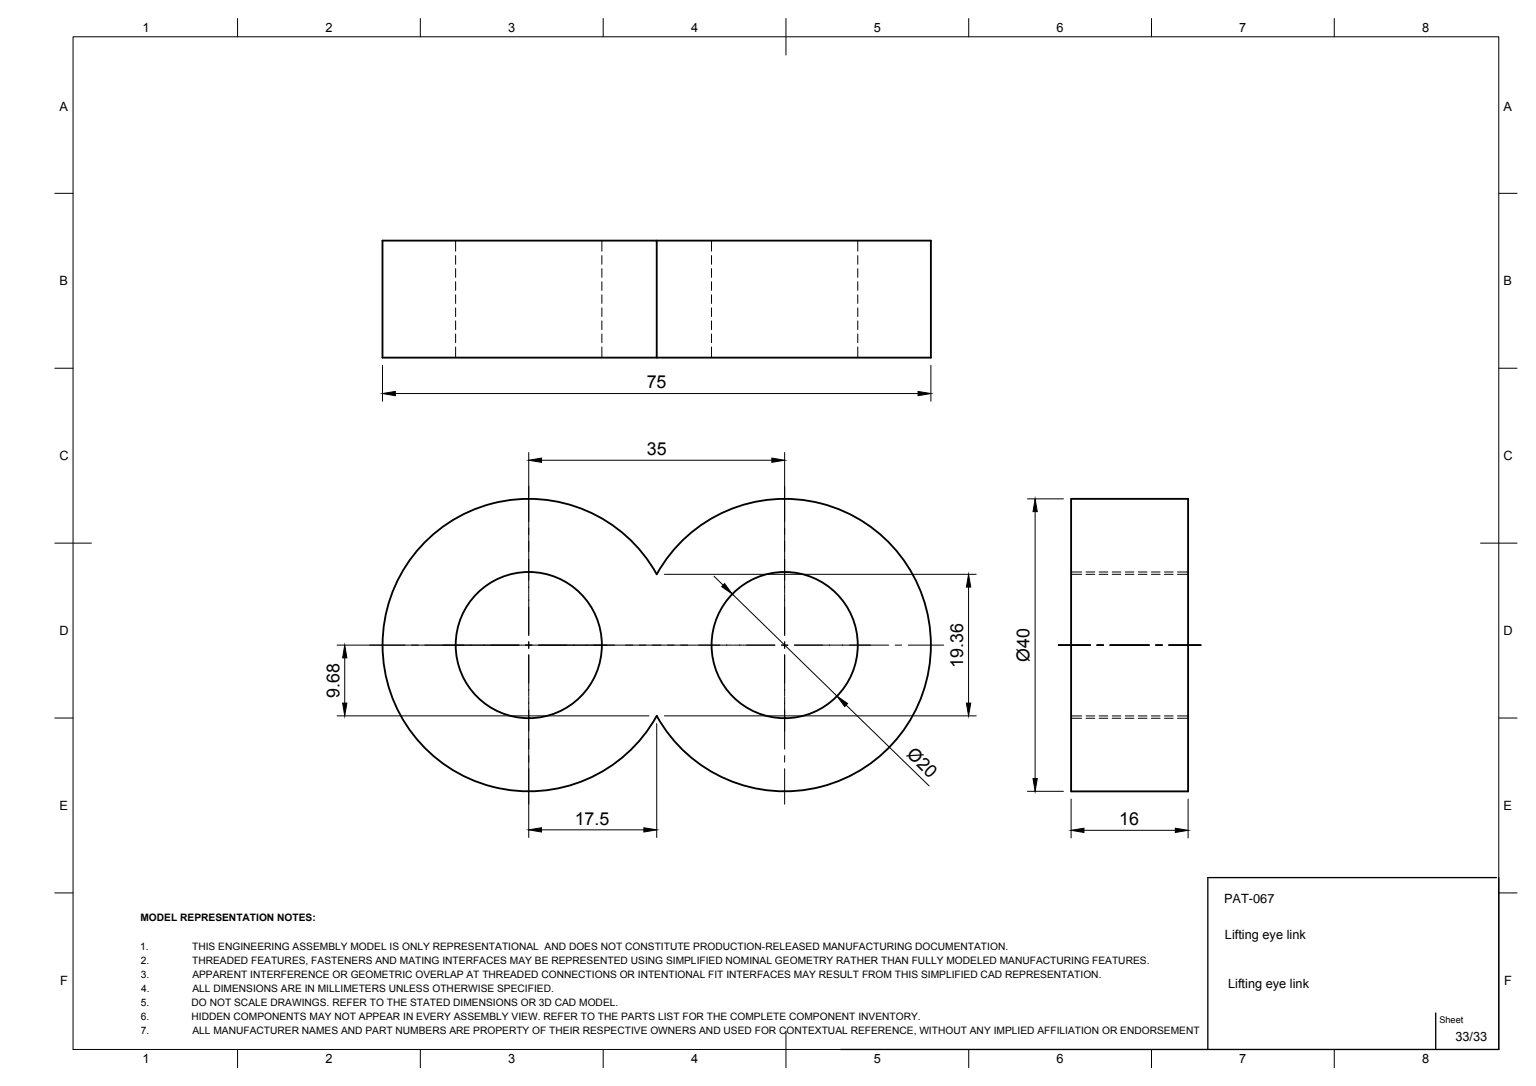
ISO-10303-21;
HEADER;
/* Generated by software containing ST-Developer
 * from STEP Tools, Inc. (www.steptools.com) 
 */

FILE_DESCRIPTION(
/* description */ ('Lifting hook block with sheave'),
/* implementation_level */ '2;1');

FILE_NAME(
/* name */ 'Lifting eye link.step',
/* time_stamp */ '2026-10-28T03:23:54-07:00',
/* author */ (''),
/* organization */ (''),
/* preprocessor_version */ 'ST-DEVELOPER v20.2',
/* originating_system */ 'Autodesk Translation Framework v15.17.0.0',
/* authorisation */ '');

FILE_SCHEMA (('AUTOMOTIVE_DESIGN { 1 0 10303 214 3 1 1 }'));
ENDSEC;

DATA;
#10=MECHANICAL_DESIGN_GEOMETRIC_PRESENTATION_REPRESENTATION('',(#388),#9391);
#320=SHAPE_REPRESENTATION_RELATIONSHIP('SRR','None',#9555,#350);
#350=ADVANCED_BREP_SHAPE_REPRESENTATION('',(#423),#9390);
#388=STYLED_ITEM('',(#9752),#423);
#423=MANIFOLD_SOLID_BREP('Body1',#4927);
#708=LINE('',#9291,#996);
#709=LINE('',#9297,#997);
#710=LINE('',#9302,#998);
#711=LINE('',#9306,#999);
#996=VECTOR('',#7519,1.);
#997=VECTOR('',#7526,1.);
#998=VECTOR('',#7531,1.);
#999=VECTOR('',#7534,1.);
#1103=CYLINDRICAL_SURFACE('',#5910,1.);
#1104=CYLINDRICAL_SURFACE('',#5913,1.);
#1105=CYLINDRICAL_SURFACE('',#5916,2.);
#1106=CYLINDRICAL_SURFACE('',#5921,2.);
#1218=FACE_BOUND('',#1909,.T.);
#1219=FACE_BOUND('',#1910,.T.);
#1220=FACE_BOUND('',#1913,.T.);
#1221=FACE_BOUND('',#1914,.T.);
#1505=FACE_OUTER_BOUND('',#1905,.T.);
#1506=FACE_OUTER_BOUND('',#1906,.T.);
#1507=FACE_OUTER_BOUND('',#1907,.T.);
#1508=FACE_OUTER_BOUND('',#1908,.T.);
#1509=FACE_OUTER_BOUND('',#1911,.T.);
#1510=FACE_OUTER_BOUND('',#1912,.T.);
#1905=EDGE_LOOP('',(#4428,#4429,#4430,#4431));
#1906=EDGE_LOOP('',(#4432,#4433,#4434,#4435));
#1907=EDGE_LOOP('',(#4436,#4437,#4438,#4439));
#1908=EDGE_LOOP('',(#4440,#4441));
#1909=EDGE_LOOP('',(#4442));
#1910=EDGE_LOOP('',(#4443));
#1911=EDGE_LOOP('',(#4444,#4445,#4446,#4447));
#1912=EDGE_LOOP('',(#4448,#4449));
#1913=EDGE_LOOP('',(#4450));
#1914=EDGE_LOOP('',(#4451));
#2200=CIRCLE('',#5911,1.);
#2201=CIRCLE('',#5912,1.);
#2202=CIRCLE('',#5914,1.);
#2203=CIRCLE('',#5915,1.);
#2204=CIRCLE('',#5917,2.);
#2205=CIRCLE('',#5918,2.);
#2206=CIRCLE('',#5920,2.);
#2207=CIRCLE('',#5922,2.);
#2611=VERTEX_POINT('',#9288);
#2612=VERTEX_POINT('',#9290);
#2613=VERTEX_POINT('',#9294);
#2614=VERTEX_POINT('',#9296);
#2615=VERTEX_POINT('',#9300);
#2616=VERTEX_POINT('',#9301);
#2617=VERTEX_POINT('',#9303);
#2618=VERTEX_POINT('',#9305);
#3218=EDGE_CURVE('',#2611,#2611,#2200,.T.);
#3219=EDGE_CURVE('',#2611,#2612,#708,.T.);
#3220=EDGE_CURVE('',#2612,#2612,#2201,.T.);
#3221=EDGE_CURVE('',#2613,#2613,#2202,.T.);
#3222=EDGE_CURVE('',#2613,#2614,#709,.T.);
#3223=EDGE_CURVE('',#2614,#2614,#2203,.T.);
#3224=EDGE_CURVE('',#2615,#2616,#710,.T.);
#3225=EDGE_CURVE('',#2615,#2617,#2204,.T.);
#3226=EDGE_CURVE('',#2618,#2617,#711,.T.);
#3227=EDGE_CURVE('',#2616,#2618,#2205,.T.);
#3228=EDGE_CURVE('',#2618,#2616,#2206,.T.);
#3229=EDGE_CURVE('',#2617,#2615,#2207,.T.);
#4428=ORIENTED_EDGE('',*,*,#3218,.F.);
#4429=ORIENTED_EDGE('',*,*,#3219,.T.);
#4430=ORIENTED_EDGE('',*,*,#3220,.F.);
#4431=ORIENTED_EDGE('',*,*,#3219,.F.);
#4432=ORIENTED_EDGE('',*,*,#3221,.F.);
#4433=ORIENTED_EDGE('',*,*,#3222,.T.);
#4434=ORIENTED_EDGE('',*,*,#3223,.F.);
#4435=ORIENTED_EDGE('',*,*,#3222,.F.);
#4436=ORIENTED_EDGE('',*,*,#3224,.F.);
#4437=ORIENTED_EDGE('',*,*,#3225,.T.);
#4438=ORIENTED_EDGE('',*,*,#3226,.F.);
#4439=ORIENTED_EDGE('',*,*,#3227,.F.);
#4440=ORIENTED_EDGE('',*,*,#3228,.T.);
#4441=ORIENTED_EDGE('',*,*,#3227,.T.);
#4442=ORIENTED_EDGE('',*,*,#3220,.T.);
#4443=ORIENTED_EDGE('',*,*,#3223,.T.);
#4444=ORIENTED_EDGE('',*,*,#3224,.T.);
#4445=ORIENTED_EDGE('',*,*,#3228,.F.);
#4446=ORIENTED_EDGE('',*,*,#3226,.T.);
#4447=ORIENTED_EDGE('',*,*,#3229,.T.);
#4448=ORIENTED_EDGE('',*,*,#3229,.F.);
#4449=ORIENTED_EDGE('',*,*,#3225,.F.);
#4450=ORIENTED_EDGE('',*,*,#3218,.T.);
#4451=ORIENTED_EDGE('',*,*,#3221,.T.);
#4596=PLANE('',#5919);
#4597=PLANE('',#5923);
#4881=ADVANCED_FACE('',(#1505),#1103,.F.);
#4882=ADVANCED_FACE('',(#1506),#1104,.F.);
#4883=ADVANCED_FACE('',(#1507),#1105,.T.);
#4884=ADVANCED_FACE('',(#1508,#1218,#1219),#4596,.T.);
#4885=ADVANCED_FACE('',(#1509),#1106,.T.);
#4886=ADVANCED_FACE('',(#1510,#1220,#1221),#4597,.F.);
#4927=CLOSED_SHELL('',(#4881,#4882,#4883,#4884,#4885,#4886));
#5909=AXIS2_PLACEMENT_3D('',#9286,#7513,#7514);
#5910=AXIS2_PLACEMENT_3D('',#9287,#7515,#7516);
#5911=AXIS2_PLACEMENT_3D('',#9289,#7517,#7518);
#5912=AXIS2_PLACEMENT_3D('',#9292,#7520,#7521);
#5913=AXIS2_PLACEMENT_3D('',#9293,#7522,#7523);
#5914=AXIS2_PLACEMENT_3D('',#9295,#7524,#7525);
#5915=AXIS2_PLACEMENT_3D('',#9298,#7527,#7528);
#5916=AXIS2_PLACEMENT_3D('',#9299,#7529,#7530);
#5917=AXIS2_PLACEMENT_3D('',#9304,#7532,#7533);
#5918=AXIS2_PLACEMENT_3D('',#9307,#7535,#7536);
#5919=AXIS2_PLACEMENT_3D('',#9308,#7537,#7538);
#5920=AXIS2_PLACEMENT_3D('',#9309,#7539,#7540);
#5921=AXIS2_PLACEMENT_3D('',#9310,#7541,#7542);
#5922=AXIS2_PLACEMENT_3D('',#9311,#7543,#7544);
#5923=AXIS2_PLACEMENT_3D('',#9312,#7545,#7546);
#7513=DIRECTION('axis',(0.,0.,1.));
#7514=DIRECTION('refdir',(1.,0.,0.));
#7515=DIRECTION('center_axis',(0.,1.,0.));
#7516=DIRECTION('ref_axis',(1.,0.,0.));
#7517=DIRECTION('center_axis',(0.,1.,0.));
#7518=DIRECTION('ref_axis',(1.,0.,0.));
#7519=DIRECTION('',(0.,1.,0.));
#7520=DIRECTION('center_axis',(0.,-1.,0.));
#7521=DIRECTION('ref_axis',(1.,0.,0.));
#7522=DIRECTION('center_axis',(0.,1.,0.));
#7523=DIRECTION('ref_axis',(1.,0.,0.));
#7524=DIRECTION('center_axis',(0.,1.,0.));
#7525=DIRECTION('ref_axis',(1.,0.,0.));
#7526=DIRECTION('',(0.,1.,0.));
#7527=DIRECTION('center_axis',(0.,-1.,0.));
#7528=DIRECTION('ref_axis',(1.,0.,0.));
#7529=DIRECTION('center_axis',(0.,1.,0.));
#7530=DIRECTION('ref_axis',(-1.83697019872103E-16,0.,1.));
#7531=DIRECTION('',(0.,1.,0.));
#7532=DIRECTION('center_axis',(0.,1.,0.));
#7533=DIRECTION('ref_axis',(1.,0.,0.));
#7534=DIRECTION('',(0.,-1.,0.));
#7535=DIRECTION('center_axis',(0.,1.,0.));
#7536=DIRECTION('ref_axis',(1.,0.,0.));
#7537=DIRECTION('center_axis',(0.,1.,0.));
#7538=DIRECTION('ref_axis',(1.,0.,0.));
#7539=DIRECTION('center_axis',(0.,1.,0.));
#7540=DIRECTION('ref_axis',(1.,0.,0.));
#7541=DIRECTION('center_axis',(0.,1.,0.));
#7542=DIRECTION('ref_axis',(-1.83697019872103E-16,0.,-1.));
#7543=DIRECTION('center_axis',(0.,1.,0.));
#7544=DIRECTION('ref_axis',(1.,0.,0.));
#7545=DIRECTION('center_axis',(0.,1.,0.));
#7546=DIRECTION('ref_axis',(1.,0.,0.));
#9286=CARTESIAN_POINT('',(0.,0.,0.));
#9287=CARTESIAN_POINT('Origin',(0.,-0.9,20.5));
#9288=CARTESIAN_POINT('',(-1.,-0.8,20.5));
#9289=CARTESIAN_POINT('Origin',(0.,-0.8,20.5));
#9290=CARTESIAN_POINT('',(-1.,0.8,20.5));
#9291=CARTESIAN_POINT('',(-1.,-0.9,20.5));
#9292=CARTESIAN_POINT('Origin',(0.,0.8,20.5));
#9293=CARTESIAN_POINT('Origin',(0.,-0.9,24.));
#9294=CARTESIAN_POINT('',(-1.,-0.8,24.));
#9295=CARTESIAN_POINT('Origin',(0.,-0.8,24.));
#9296=CARTESIAN_POINT('',(-1.,0.8,24.));
#9297=CARTESIAN_POINT('',(-1.,-0.9,24.));
#9298=CARTESIAN_POINT('Origin',(0.,0.8,24.));
#9299=CARTESIAN_POINT('Origin',(0.,-0.8,24.));
#9300=CARTESIAN_POINT('',(-0.968245836551854,-0.8,22.25));
#9301=CARTESIAN_POINT('',(-0.968245836551854,0.8,22.25));
#9302=CARTESIAN_POINT('',(-0.968245836551854,-0.8,22.25));
#9303=CARTESIAN_POINT('',(0.968245836551854,-0.8,22.25));
#9304=CARTESIAN_POINT('Origin',(0.,-0.8,24.));
#9305=CARTESIAN_POINT('',(0.968245836551854,0.8,22.25));
#9306=CARTESIAN_POINT('',(0.968245836551854,-0.8,22.25));
#9307=CARTESIAN_POINT('Origin',(0.,0.8,24.));
#9308=CARTESIAN_POINT('Origin',(0.,0.8,20.5));
#9309=CARTESIAN_POINT('Origin',(0.,0.8,20.5));
#9310=CARTESIAN_POINT('Origin',(0.,-0.8,20.5));
#9311=CARTESIAN_POINT('Origin',(0.,-0.8,20.5));
#9312=CARTESIAN_POINT('Origin',(0.,-0.8,20.5));
#9353=UNCERTAINTY_MEASURE_WITH_UNIT(LENGTH_MEASURE(0.001),#9392,
'DISTANCE_ACCURACY_VALUE',
'Maximum model space distance between geometric entities at asserted c
onnectivities');
#9354=UNCERTAINTY_MEASURE_WITH_UNIT(LENGTH_MEASURE(0.001),#9392,
'DISTANCE_ACCURACY_VALUE',
'Maximum model space distance between geometric entities at asserted c
onnectivities');
#9390=(
GEOMETRIC_REPRESENTATION_CONTEXT(3)
GLOBAL_UNCERTAINTY_ASSIGNED_CONTEXT((#9353))
GLOBAL_UNIT_ASSIGNED_CONTEXT((#9392,#9394,#9395))
REPRESENTATION_CONTEXT('','3D')
);
#9391=(
GEOMETRIC_REPRESENTATION_CONTEXT(3)
GLOBAL_UNCERTAINTY_ASSIGNED_CONTEXT((#9354))
GLOBAL_UNIT_ASSIGNED_CONTEXT((#9392,#9394,#9395))
REPRESENTATION_CONTEXT('','3D')
);
#9392=(
LENGTH_UNIT()
NAMED_UNIT(*)
SI_UNIT(.CENTI.,.METRE.)
);
#9394=(
NAMED_UNIT(*)
PLANE_ANGLE_UNIT()
SI_UNIT($,.RADIAN.)
);
#9395=(
NAMED_UNIT(*)
SI_UNIT($,.STERADIAN.)
SOLID_ANGLE_UNIT()
);
#9431=SHAPE_DEFINITION_REPRESENTATION(#9514,#9555);
#9514=PRODUCT_DEFINITION_SHAPE('',$,#9592);
#9555=SHAPE_REPRESENTATION('',(#5909),#9390);
#9556=PRODUCT_DEFINITION_CONTEXT('part definition',#9666,'design');
#9592=PRODUCT_DEFINITION('Lifting eye link','Lifting eye link',#9628,#9556);
#9628=PRODUCT_DEFINITION_FORMATION('',$,#9703);
#9666=APPLICATION_CONTEXT(
'Core Data for Automotive Mechanical Design Process');
#9667=PRODUCT_CONTEXT('part definition',#9666,'mechanical');
#9703=PRODUCT('Lifting eye link','Lifting eye link','Lifting eye link',
(#9667));
#9746=COLOUR_RGB('Sky Blue',0.24,0.69,0.87);
#9747=FILL_AREA_STYLE_COLOUR('',#9746);
#9748=FILL_AREA_STYLE('',(#9747));
#9749=SURFACE_STYLE_FILL_AREA(#9748);
#9750=SURFACE_SIDE_STYLE('',(#9749));
#9751=SURFACE_STYLE_USAGE(.BOTH.,#9750);
#9752=PRESENTATION_STYLE_ASSIGNMENT((#9751));
ENDSEC;
END-ISO-10303-21;
